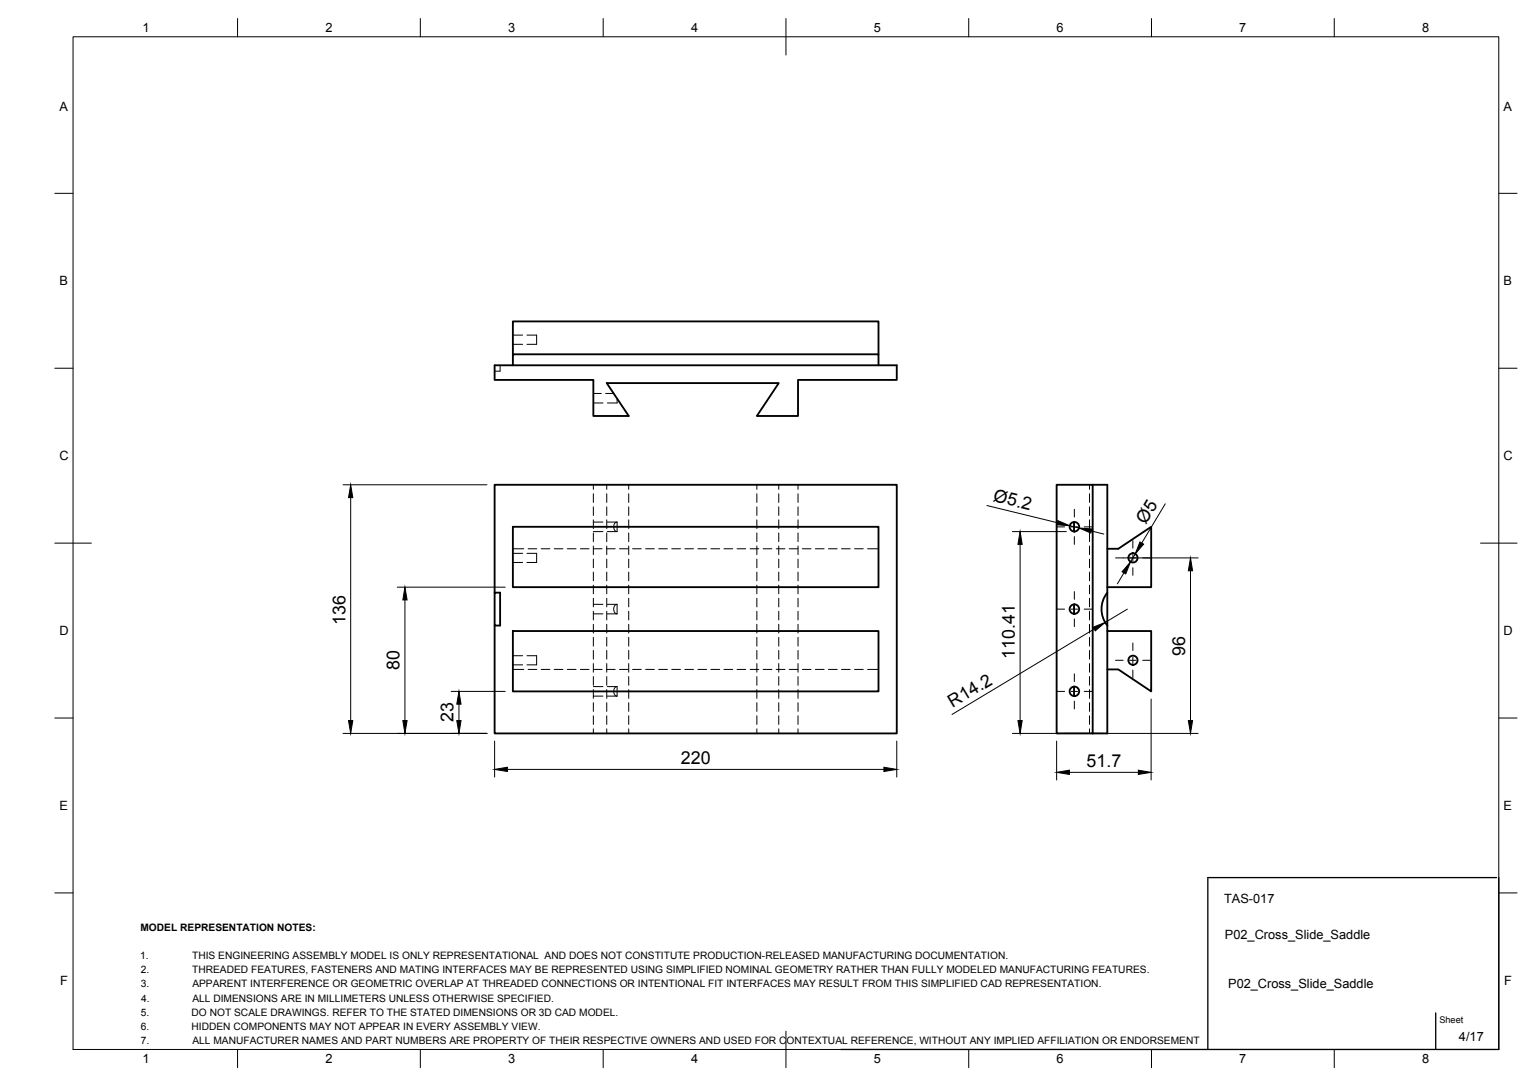
ISO-10303-21;
HEADER;
/* Generated by software containing ST-Developer
 * from STEP Tools, Inc. (www.steptools.com) 
 */

FILE_DESCRIPTION(
/* description */ ('STEP AP203'),
/* implementation_level */ '2;1');

FILE_NAME(
/* name */ 'P02_Cross_Slide_Saddle.step',
/* time_stamp */ '2026-11-15T15:04:01-08:00',
/* author */ (''),
/* organization */ (''),
/* preprocessor_version */ 'ST-DEVELOPER v20.2',
/* originating_system */ 'Autodesk Translation Framework v15.17.0.0',
/* authorisation */ '');

FILE_SCHEMA (('AUTOMOTIVE_DESIGN { 1 0 10303 214 3 1 1 }'));
ENDSEC;

DATA;
#10=MECHANICAL_DESIGN_GEOMETRIC_PRESENTATION_REPRESENTATION('',(#279,#280,#281),#16598);
#195=ELLIPSE('',#10144,3.12481110540129,2.59999999999927);
#196=ELLIPSE('',#10146,3.12481110540129,2.59999999999927);
#197=ELLIPSE('',#10149,3.12481110540191,2.59999999999976);
#198=ELLIPSE('',#10151,3.12481110540191,2.59999999999976);
#199=ELLIPSE('',#10154,3.1248111054022,2.60000000000004);
#200=ELLIPSE('',#10156,3.1248111054022,2.60000000000004);
#205=SHAPE_REPRESENTATION_RELATIONSHIP('SRR','None',#16699,#229);
#229=ADVANCED_BREP_SHAPE_REPRESENTATION('',(#253),#16575);
#253=MANIFOLD_SOLID_BREP('Body1',#9788);
#279=STYLED_ITEM('',(#16828),#9306);
#280=STYLED_ITEM('',(#16828),#9312);
#281=STYLED_ITEM('',(#16829),#253);
#310=FACE_BOUND('',#1521,.T.);
#311=FACE_BOUND('',#1522,.T.);
#312=FACE_BOUND('',#1524,.T.);
#313=FACE_BOUND('',#1525,.T.);
#314=FACE_BOUND('',#1526,.T.);
#315=FACE_BOUND('',#1535,.T.);
#316=FACE_BOUND('',#1536,.T.);
#317=FACE_BOUND('',#1537,.T.);
#318=FACE_BOUND('',#1547,.T.);
#319=FACE_BOUND('',#1554,.T.);
#474=PLANE('',#10157);
#475=PLANE('',#10158);
#476=PLANE('',#10159);
#477=PLANE('',#10160);
#478=PLANE('',#10161);
#479=PLANE('',#10162);
#480=PLANE('',#10163);
#481=PLANE('',#10164);
#482=PLANE('',#10165);
#483=PLANE('',#10166);
#484=PLANE('',#10167);
#485=PLANE('',#10168);
#486=PLANE('',#10169);
#487=PLANE('',#10170);
#488=PLANE('',#10171);
#489=PLANE('',#10172);
#490=PLANE('',#10173);
#491=PLANE('',#10174);
#492=PLANE('',#10175);
#493=PLANE('',#10176);
#494=PLANE('',#10177);
#495=PLANE('',#10178);
#496=PLANE('',#10179);
#497=PLANE('',#10180);
#498=PLANE('',#10181);
#499=PLANE('',#10182);
#500=PLANE('',#10183);
#501=PLANE('',#10184);
#502=PLANE('',#10185);
#503=PLANE('',#10186);
#504=PLANE('',#10187);
#505=PLANE('',#10188);
#959=FACE_OUTER_BOUND('',#1514,.T.);
#960=FACE_OUTER_BOUND('',#1515,.T.);
#961=FACE_OUTER_BOUND('',#1516,.T.);
#962=FACE_OUTER_BOUND('',#1517,.T.);
#963=FACE_OUTER_BOUND('',#1518,.T.);
#964=FACE_OUTER_BOUND('',#1519,.T.);
#965=FACE_OUTER_BOUND('',#1520,.T.);
#966=FACE_OUTER_BOUND('',#1523,.T.);
#967=FACE_OUTER_BOUND('',#1527,.T.);
#968=FACE_OUTER_BOUND('',#1528,.T.);
#969=FACE_OUTER_BOUND('',#1529,.T.);
#970=FACE_OUTER_BOUND('',#1530,.T.);
#971=FACE_OUTER_BOUND('',#1531,.T.);
#972=FACE_OUTER_BOUND('',#1532,.T.);
#973=FACE_OUTER_BOUND('',#1533,.T.);
#974=FACE_OUTER_BOUND('',#1534,.T.);
#975=FACE_OUTER_BOUND('',#1538,.T.);
#976=FACE_OUTER_BOUND('',#1539,.T.);
#977=FACE_OUTER_BOUND('',#1540,.T.);
#978=FACE_OUTER_BOUND('',#1541,.T.);
#979=FACE_OUTER_BOUND('',#1542,.T.);
#980=FACE_OUTER_BOUND('',#1543,.T.);
#981=FACE_OUTER_BOUND('',#1544,.T.);
#982=FACE_OUTER_BOUND('',#1545,.T.);
#983=FACE_OUTER_BOUND('',#1546,.T.);
#984=FACE_OUTER_BOUND('',#1548,.T.);
#985=FACE_OUTER_BOUND('',#1549,.T.);
#986=FACE_OUTER_BOUND('',#1550,.T.);
#987=FACE_OUTER_BOUND('',#1551,.T.);
#988=FACE_OUTER_BOUND('',#1552,.T.);
#989=FACE_OUTER_BOUND('',#1553,.T.);
#990=FACE_OUTER_BOUND('',#1555,.T.);
#991=FACE_OUTER_BOUND('',#1556,.T.);
#992=FACE_OUTER_BOUND('',#1557,.T.);
#993=FACE_OUTER_BOUND('',#1558,.T.);
#994=FACE_OUTER_BOUND('',#1559,.T.);
#995=FACE_OUTER_BOUND('',#1560,.T.);
#996=FACE_OUTER_BOUND('',#1561,.T.);
#1514=EDGE_LOOP('',(#6849,#6850,#6851,#6852));
#1515=EDGE_LOOP('',(#6853,#6854,#6855,#6856));
#1516=EDGE_LOOP('',(#6857,#6858,#6859,#6860));
#1517=EDGE_LOOP('',(#6861,#6862,#6863,#6864,#6865,#6866));
#1518=EDGE_LOOP('',(#6867,#6868,#6869,#6870,#6871,#6872));
#1519=EDGE_LOOP('',(#6873,#6874,#6875,#6876,#6877,#6878));
#1520=EDGE_LOOP('',(#6879,#6880,#6881,#6882,#6883,#6884,#6885,#6886));
#1521=EDGE_LOOP('',(#6887,#6888,#6889,#6890));
#1522=EDGE_LOOP('',(#6891,#6892,#6893,#6894));
#1523=EDGE_LOOP('',(#6895,#6896,#6897,#6898));
#1524=EDGE_LOOP('',(#6899,#6900,#6901));
#1525=EDGE_LOOP('',(#6902,#6903,#6904));
#1526=EDGE_LOOP('',(#6905,#6906,#6907));
#1527=EDGE_LOOP('',(#6908,#6909,#6910,#6911));
#1528=EDGE_LOOP('',(#6912,#6913,#6914,#6915));
#1529=EDGE_LOOP('',(#6916,#6917,#6918,#6919));
#1530=EDGE_LOOP('',(#6920,#6921,#6922,#6923));
#1531=EDGE_LOOP('',(#6924,#6925,#6926,#6927));
#1532=EDGE_LOOP('',(#6928,#6929,#6930,#6931));
#1533=EDGE_LOOP('',(#6932,#6933,#6934,#6935));
#1534=EDGE_LOOP('',(#6936,#6937,#6938,#6939));
#1535=EDGE_LOOP('',(#6940));
#1536=EDGE_LOOP('',(#6941));
#1537=EDGE_LOOP('',(#6942));
#1538=EDGE_LOOP('',(#6943,#6944,#6945,#6946));
#1539=EDGE_LOOP('',(#6947,#6948,#6949,#6950,#6951,#6952));
#1540=EDGE_LOOP('',(#6953,#6954,#6955,#6956,#6957,#6958,#6959,#6960,#6961,
#6962,#6963,#6964));
#1541=EDGE_LOOP('',(#6965,#6966,#6967,#6968,#6969,#6970,#6971,#6972,#6973,
#6974,#6975,#6976));
#1542=EDGE_LOOP('',(#6977,#6978,#6979,#6980));
#1543=EDGE_LOOP('',(#6981,#6982,#6983,#6984));
#1544=EDGE_LOOP('',(#6985,#6986,#6987,#6988));
#1545=EDGE_LOOP('',(#6989,#6990,#6991,#6992));
#1546=EDGE_LOOP('',(#6993,#6994,#6995,#6996,#6997));
#1547=EDGE_LOOP('',(#6998));
#1548=EDGE_LOOP('',(#6999,#7000,#7001,#7002,#7003));
#1549=EDGE_LOOP('',(#7004,#7005,#7006,#7007));
#1550=EDGE_LOOP('',(#7008,#7009,#7010,#7011));
#1551=EDGE_LOOP('',(#7012,#7013,#7014,#7015));
#1552=EDGE_LOOP('',(#7016,#7017,#7018,#7019));
#1553=EDGE_LOOP('',(#7020,#7021,#7022,#7023,#7024));
#1554=EDGE_LOOP('',(#7025));
#1555=EDGE_LOOP('',(#7026,#7027,#7028,#7029,#7030));
#1556=EDGE_LOOP('',(#7031,#7032));
#1557=EDGE_LOOP('',(#7033,#7034));
#1558=EDGE_LOOP('',(#7035,#7036));
#1559=EDGE_LOOP('',(#7037));
#1560=EDGE_LOOP('',(#7038));
#1561=EDGE_LOOP('',(#7039,#7040));
#2256=LINE('',#13946,#3304);
#2257=LINE('',#13949,#3305);
#2258=LINE('',#13954,#3306);
#2259=LINE('',#13960,#3307);
#2260=LINE('',#13966,#3308);
#2261=LINE('',#13976,#3309);
#2262=LINE('',#13986,#3310);
#2263=LINE('',#13993,#3311);
#2264=LINE('',#13995,#3312);
#2265=LINE('',#13997,#3313);
#2266=LINE('',#13999,#3314);
#2267=LINE('',#14001,#3315);
#2268=LINE('',#14002,#3316);
#2269=LINE('',#14005,#3317);
#2270=LINE('',#14007,#3318);
#2271=LINE('',#14009,#3319);
#2272=LINE('',#14010,#3320);
#2273=LINE('',#14013,#3321);
#2274=LINE('',#14015,#3322);
#2275=LINE('',#14017,#3323);
#2276=LINE('',#14018,#3324);
#2277=LINE('',#14022,#3325);
#2278=LINE('',#14024,#3326);
#2279=LINE('',#14026,#3327);
#2280=LINE('',#14027,#3328);
#2281=LINE('',#14028,#3329);
#2282=LINE('',#14029,#3330);
#2283=LINE('',#14030,#3331);
#2284=LINE('',#14033,#3332);
#2285=LINE('',#14035,#3333);
#2286=LINE('',#14036,#3334);
#2287=LINE('',#14039,#3335);
#2288=LINE('',#14041,#3336);
#2289=LINE('',#14042,#3337);
#2290=LINE('',#14045,#3338);
#2291=LINE('',#14047,#3339);
#2292=LINE('',#14048,#3340);
#2293=LINE('',#14051,#3341);
#2294=LINE('',#14053,#3342);
#2295=LINE('',#14054,#3343);
#2296=LINE('',#14057,#3344);
#2297=LINE('',#14059,#3345);
#2298=LINE('',#14060,#3346);
#2299=LINE('',#14062,#3347);
#2300=LINE('',#14063,#3348);
#2301=LINE('',#14066,#3349);
#2302=LINE('',#14068,#3350);
#2303=LINE('',#14069,#3351);
#2304=LINE('',#14072,#3352);
#2305=LINE('',#14074,#3353);
#2306=LINE('',#14075,#3354);
#2307=LINE('',#14078,#3355);
#2308=LINE('',#14080,#3356);
#2309=LINE('',#14081,#3357);
#2310=LINE('',#14083,#3358);
#2311=LINE('',#14084,#3359);
#2312=LINE('',#14089,#3360);
#2313=LINE('',#14091,#3361);
#2314=LINE('',#14092,#3362);
#2315=LINE('',#14095,#3363);
#2316=LINE('',#14097,#3364);
#2317=LINE('',#14098,#3365);
#2318=LINE('',#14101,#3366);
#2319=LINE('',#14103,#3367);
#2320=LINE('',#14104,#3368);
#2321=LINE('',#14106,#3369);
#2322=LINE('',#14107,#3370);
#2323=LINE('',#14112,#3371);
#2324=LINE('',#14114,#3372);
#2325=LINE('',#14115,#3373);
#2326=LINE('',#14118,#3374);
#2327=LINE('',#14120,#3375);
#2328=LINE('',#14121,#3376);
#2329=LINE('',#14124,#3377);
#2330=LINE('',#14126,#3378);
#2331=LINE('',#14127,#3379);
#2332=LINE('',#14129,#3380);
#2333=LINE('',#14130,#3381);
#3304=VECTOR('',#11166,1000.);
#3305=VECTOR('',#11169,1000.);
#3306=VECTOR('',#11174,2.5);
#3307=VECTOR('',#11181,2.5);
#3308=VECTOR('',#11188,2.6);
#3309=VECTOR('',#11199,2.6);
#3310=VECTOR('',#11210,2.6);
#3311=VECTOR('',#11219,1000.);
#3312=VECTOR('',#11220,1000.);
#3313=VECTOR('',#11221,1000.);
#3314=VECTOR('',#11222,1000.);
#3315=VECTOR('',#11223,1000.);
#3316=VECTOR('',#11224,1000.);
#3317=VECTOR('',#11225,1000.);
#3318=VECTOR('',#11226,1000.);
#3319=VECTOR('',#11227,1000.);
#3320=VECTOR('',#11228,1000.);
#3321=VECTOR('',#11229,1000.);
#3322=VECTOR('',#11230,1000.);
#3323=VECTOR('',#11231,1000.);
#3324=VECTOR('',#11232,1000.);
#3325=VECTOR('',#11235,1000.);
#3326=VECTOR('',#11236,1000.);
#3327=VECTOR('',#11237,1000.);
#3328=VECTOR('',#11238,1000.);
#3329=VECTOR('',#11239,1000.);
#3330=VECTOR('',#11240,1000.);
#3331=VECTOR('',#11241,1000.);
#3332=VECTOR('',#11244,1000.);
#3333=VECTOR('',#11245,1000.);
#3334=VECTOR('',#11246,1000.);
#3335=VECTOR('',#11249,1000.);
#3336=VECTOR('',#11250,1000.);
#3337=VECTOR('',#11251,1000.);
#3338=VECTOR('',#11254,1000.);
#3339=VECTOR('',#11255,1000.);
#3340=VECTOR('',#11256,1000.);
#3341=VECTOR('',#11259,1000.);
#3342=VECTOR('',#11260,1000.);
#3343=VECTOR('',#11261,1000.);
#3344=VECTOR('',#11264,1000.);
#3345=VECTOR('',#11265,1000.);
#3346=VECTOR('',#11266,1000.);
#3347=VECTOR('',#11269,1000.);
#3348=VECTOR('',#11270,1000.);
#3349=VECTOR('',#11273,1000.);
#3350=VECTOR('',#11274,1000.);
#3351=VECTOR('',#11275,1000.);
#3352=VECTOR('',#11278,1000.);
#3353=VECTOR('',#11279,1000.);
#3354=VECTOR('',#11280,1000.);
#3355=VECTOR('',#11283,1000.);
#3356=VECTOR('',#11284,1000.);
#3357=VECTOR('',#11285,1000.);
#3358=VECTOR('',#11288,1000.);
#3359=VECTOR('',#11289,1000.);
#3360=VECTOR('',#11296,1000.);
#3361=VECTOR('',#11297,1000.);
#3362=VECTOR('',#11298,1000.);
#3363=VECTOR('',#11301,1000.);
#3364=VECTOR('',#11302,1000.);
#3365=VECTOR('',#11303,1000.);
#3366=VECTOR('',#11306,1000.);
#3367=VECTOR('',#11307,1000.);
#3368=VECTOR('',#11308,1000.);
#3369=VECTOR('',#11311,1000.);
#3370=VECTOR('',#11312,1000.);
#3371=VECTOR('',#11319,1000.);
#3372=VECTOR('',#11320,1000.);
#3373=VECTOR('',#11321,1000.);
#3374=VECTOR('',#11324,1000.);
#3375=VECTOR('',#11325,1000.);
#3376=VECTOR('',#11326,1000.);
#3377=VECTOR('',#11329,1000.);
#3378=VECTOR('',#11330,1000.);
#3379=VECTOR('',#11331,1000.);
#3380=VECTOR('',#11334,1000.);
#3381=VECTOR('',#11335,1000.);
#4238=CIRCLE('',#10134,14.2);
#4239=CIRCLE('',#10135,14.2);
#4240=CIRCLE('',#10137,2.5);
#4241=CIRCLE('',#10138,2.5);
#4242=CIRCLE('',#10140,2.5);
#4243=CIRCLE('',#10141,2.5);
#4244=CIRCLE('',#10143,2.6);
#4245=CIRCLE('',#10145,2.6);
#4246=CIRCLE('',#10148,2.6);
#4247=CIRCLE('',#10150,2.6);
#4248=CIRCLE('',#10153,2.6);
#4249=CIRCLE('',#10155,2.6);
#4539=VERTEX_POINT('',#13942);
#4540=VERTEX_POINT('',#13943);
#4541=VERTEX_POINT('',#13945);
#4542=VERTEX_POINT('',#13947);
#4543=VERTEX_POINT('',#13951);
#4544=VERTEX_POINT('',#13953);
#4545=VERTEX_POINT('',#13957);
#4546=VERTEX_POINT('',#13959);
#4547=VERTEX_POINT('',#13963);
#4548=VERTEX_POINT('',#13965);
#4549=VERTEX_POINT('',#13967);
#4550=VERTEX_POINT('',#13969);
#4551=VERTEX_POINT('',#13973);
#4552=VERTEX_POINT('',#13975);
#4553=VERTEX_POINT('',#13977);
#4554=VERTEX_POINT('',#13979);
#4555=VERTEX_POINT('',#13983);
#4556=VERTEX_POINT('',#13985);
#4557=VERTEX_POINT('',#13987);
#4558=VERTEX_POINT('',#13989);
#4559=VERTEX_POINT('',#13994);
#4560=VERTEX_POINT('',#13996);
#4561=VERTEX_POINT('',#13998);
#4562=VERTEX_POINT('',#14000);
#4563=VERTEX_POINT('',#14003);
#4564=VERTEX_POINT('',#14004);
#4565=VERTEX_POINT('',#14006);
#4566=VERTEX_POINT('',#14008);
#4567=VERTEX_POINT('',#14011);
#4568=VERTEX_POINT('',#14012);
#4569=VERTEX_POINT('',#14014);
#4570=VERTEX_POINT('',#14016);
#4571=VERTEX_POINT('',#14020);
#4572=VERTEX_POINT('',#14021);
#4573=VERTEX_POINT('',#14023);
#4574=VERTEX_POINT('',#14025);
#4575=VERTEX_POINT('',#14032);
#4576=VERTEX_POINT('',#14034);
#4577=VERTEX_POINT('',#14038);
#4578=VERTEX_POINT('',#14040);
#4579=VERTEX_POINT('',#14044);
#4580=VERTEX_POINT('',#14046);
#4581=VERTEX_POINT('',#14050);
#4582=VERTEX_POINT('',#14052);
#4583=VERTEX_POINT('',#14056);
#4584=VERTEX_POINT('',#14058);
#4585=VERTEX_POINT('',#14065);
#4586=VERTEX_POINT('',#14067);
#4587=VERTEX_POINT('',#14071);
#4588=VERTEX_POINT('',#14073);
#4589=VERTEX_POINT('',#14077);
#4590=VERTEX_POINT('',#14079);
#4591=VERTEX_POINT('',#14088);
#4592=VERTEX_POINT('',#14090);
#4593=VERTEX_POINT('',#14094);
#4594=VERTEX_POINT('',#14096);
#4595=VERTEX_POINT('',#14100);
#4596=VERTEX_POINT('',#14102);
#4597=VERTEX_POINT('',#14111);
#4598=VERTEX_POINT('',#14113);
#4599=VERTEX_POINT('',#14117);
#4600=VERTEX_POINT('',#14119);
#4601=VERTEX_POINT('',#14123);
#4602=VERTEX_POINT('',#14125);
#5437=EDGE_CURVE('',#4539,#4540,#4238,.T.);
#5438=EDGE_CURVE('',#4540,#4541,#2256,.T.);
#5439=EDGE_CURVE('',#4542,#4541,#4239,.T.);
#5440=EDGE_CURVE('',#4542,#4539,#2257,.T.);
#5441=EDGE_CURVE('',#4543,#4543,#4240,.T.);
#5442=EDGE_CURVE('',#4543,#4544,#2258,.T.);
#5443=EDGE_CURVE('',#4544,#4544,#4241,.T.);
#5444=EDGE_CURVE('',#4545,#4545,#4242,.T.);
#5445=EDGE_CURVE('',#4545,#4546,#2259,.T.);
#5446=EDGE_CURVE('',#4546,#4546,#4243,.T.);
#5447=EDGE_CURVE('',#4547,#4547,#4244,.T.);
#5448=EDGE_CURVE('',#4547,#4548,#2260,.T.);
#5449=EDGE_CURVE('',#4548,#4549,#195,.T.);
#5450=EDGE_CURVE('',#4550,#4549,#4245,.T.);
#5451=EDGE_CURVE('',#4550,#4548,#196,.T.);
#5452=EDGE_CURVE('',#4551,#4551,#4246,.T.);
#5453=EDGE_CURVE('',#4551,#4552,#2261,.T.);
#5454=EDGE_CURVE('',#4552,#4553,#197,.T.);
#5455=EDGE_CURVE('',#4554,#4553,#4247,.T.);
#5456=EDGE_CURVE('',#4554,#4552,#198,.T.);
#5457=EDGE_CURVE('',#4555,#4555,#4248,.T.);
#5458=EDGE_CURVE('',#4555,#4556,#2262,.T.);
#5459=EDGE_CURVE('',#4556,#4557,#199,.T.);
#5460=EDGE_CURVE('',#4558,#4557,#4249,.T.);
#5461=EDGE_CURVE('',#4558,#4556,#200,.T.);
#5462=EDGE_CURVE('',#4541,#4542,#2263,.T.);
#5463=EDGE_CURVE('',#4540,#4559,#2264,.T.);
#5464=EDGE_CURVE('',#4559,#4560,#2265,.T.);
#5465=EDGE_CURVE('',#4561,#4560,#2266,.T.);
#5466=EDGE_CURVE('',#4562,#4561,#2267,.T.);
#5467=EDGE_CURVE('',#4562,#4539,#2268,.T.);
#5468=EDGE_CURVE('',#4563,#4564,#2269,.T.);
#5469=EDGE_CURVE('',#4563,#4565,#2270,.T.);
#5470=EDGE_CURVE('',#4565,#4566,#2271,.T.);
#5471=EDGE_CURVE('',#4564,#4566,#2272,.T.);
#5472=EDGE_CURVE('',#4567,#4568,#2273,.T.);
#5473=EDGE_CURVE('',#4569,#4567,#2274,.T.);
#5474=EDGE_CURVE('',#4569,#4570,#2275,.T.);
#5475=EDGE_CURVE('',#4570,#4568,#2276,.T.);
#5476=EDGE_CURVE('',#4571,#4572,#2277,.T.);
#5477=EDGE_CURVE('',#4573,#4572,#2278,.T.);
#5478=EDGE_CURVE('',#4574,#4573,#2279,.T.);
#5479=EDGE_CURVE('',#4574,#4571,#2280,.T.);
#5480=EDGE_CURVE('',#4557,#4558,#2281,.T.);
#5481=EDGE_CURVE('',#4549,#4550,#2282,.T.);
#5482=EDGE_CURVE('',#4553,#4554,#2283,.T.);
#5483=EDGE_CURVE('',#4560,#4575,#2284,.T.);
#5484=EDGE_CURVE('',#4576,#4575,#2285,.T.);
#5485=EDGE_CURVE('',#4561,#4576,#2286,.T.);
#5486=EDGE_CURVE('',#4575,#4577,#2287,.T.);
#5487=EDGE_CURVE('',#4578,#4577,#2288,.T.);
#5488=EDGE_CURVE('',#4576,#4578,#2289,.T.);
#5489=EDGE_CURVE('',#4577,#4579,#2290,.T.);
#5490=EDGE_CURVE('',#4580,#4579,#2291,.T.);
#5491=EDGE_CURVE('',#4578,#4580,#2292,.T.);
#5492=EDGE_CURVE('',#4579,#4581,#2293,.T.);
#5493=EDGE_CURVE('',#4582,#4581,#2294,.T.);
#5494=EDGE_CURVE('',#4580,#4582,#2295,.T.);
#5495=EDGE_CURVE('',#4581,#4583,#2296,.T.);
#5496=EDGE_CURVE('',#4584,#4583,#2297,.T.);
#5497=EDGE_CURVE('',#4582,#4584,#2298,.T.);
#5498=EDGE_CURVE('',#4583,#4571,#2299,.T.);
#5499=EDGE_CURVE('',#4584,#4574,#2300,.T.);
#5500=EDGE_CURVE('',#4572,#4585,#2301,.T.);
#5501=EDGE_CURVE('',#4586,#4585,#2302,.T.);
#5502=EDGE_CURVE('',#4573,#4586,#2303,.T.);
#5503=EDGE_CURVE('',#4585,#4587,#2304,.T.);
#5504=EDGE_CURVE('',#4588,#4587,#2305,.T.);
#5505=EDGE_CURVE('',#4586,#4588,#2306,.T.);
#5506=EDGE_CURVE('',#4587,#4589,#2307,.T.);
#5507=EDGE_CURVE('',#4590,#4589,#2308,.T.);
#5508=EDGE_CURVE('',#4588,#4590,#2309,.T.);
#5509=EDGE_CURVE('',#4590,#4562,#2310,.T.);
#5510=EDGE_CURVE('',#4589,#4559,#2311,.T.);
#5511=EDGE_CURVE('',#4566,#4591,#2312,.T.);
#5512=EDGE_CURVE('',#4592,#4591,#2313,.T.);
#5513=EDGE_CURVE('',#4564,#4592,#2314,.T.);
#5514=EDGE_CURVE('',#4591,#4593,#2315,.T.);
#5515=EDGE_CURVE('',#4594,#4593,#2316,.T.);
#5516=EDGE_CURVE('',#4592,#4594,#2317,.T.);
#5517=EDGE_CURVE('',#4593,#4595,#2318,.T.);
#5518=EDGE_CURVE('',#4596,#4595,#2319,.T.);
#5519=EDGE_CURVE('',#4594,#4596,#2320,.T.);
#5520=EDGE_CURVE('',#4595,#4565,#2321,.T.);
#5521=EDGE_CURVE('',#4596,#4563,#2322,.T.);
#5522=EDGE_CURVE('',#4597,#4570,#2323,.T.);
#5523=EDGE_CURVE('',#4598,#4569,#2324,.T.);
#5524=EDGE_CURVE('',#4598,#4597,#2325,.T.);
#5525=EDGE_CURVE('',#4568,#4599,#2326,.T.);
#5526=EDGE_CURVE('',#4600,#4599,#2327,.T.);
#5527=EDGE_CURVE('',#4567,#4600,#2328,.T.);
#5528=EDGE_CURVE('',#4599,#4601,#2329,.T.);
#5529=EDGE_CURVE('',#4602,#4601,#2330,.T.);
#5530=EDGE_CURVE('',#4600,#4602,#2331,.T.);
#5531=EDGE_CURVE('',#4601,#4597,#2332,.T.);
#5532=EDGE_CURVE('',#4602,#4598,#2333,.T.);
#6849=ORIENTED_EDGE('',*,*,#5437,.T.);
#6850=ORIENTED_EDGE('',*,*,#5438,.T.);
#6851=ORIENTED_EDGE('',*,*,#5439,.F.);
#6852=ORIENTED_EDGE('',*,*,#5440,.T.);
#6853=ORIENTED_EDGE('',*,*,#5441,.T.);
#6854=ORIENTED_EDGE('',*,*,#5442,.T.);
#6855=ORIENTED_EDGE('',*,*,#5443,.F.);
#6856=ORIENTED_EDGE('',*,*,#5442,.F.);
#6857=ORIENTED_EDGE('',*,*,#5444,.F.);
#6858=ORIENTED_EDGE('',*,*,#5445,.T.);
#6859=ORIENTED_EDGE('',*,*,#5446,.F.);
#6860=ORIENTED_EDGE('',*,*,#5445,.F.);
#6861=ORIENTED_EDGE('',*,*,#5447,.T.);
#6862=ORIENTED_EDGE('',*,*,#5448,.T.);
#6863=ORIENTED_EDGE('',*,*,#5449,.T.);
#6864=ORIENTED_EDGE('',*,*,#5450,.F.);
#6865=ORIENTED_EDGE('',*,*,#5451,.T.);
#6866=ORIENTED_EDGE('',*,*,#5448,.F.);
#6867=ORIENTED_EDGE('',*,*,#5452,.T.);
#6868=ORIENTED_EDGE('',*,*,#5453,.T.);
#6869=ORIENTED_EDGE('',*,*,#5454,.T.);
#6870=ORIENTED_EDGE('',*,*,#5455,.F.);
#6871=ORIENTED_EDGE('',*,*,#5456,.T.);
#6872=ORIENTED_EDGE('',*,*,#5453,.F.);
#6873=ORIENTED_EDGE('',*,*,#5457,.T.);
#6874=ORIENTED_EDGE('',*,*,#5458,.T.);
#6875=ORIENTED_EDGE('',*,*,#5459,.T.);
#6876=ORIENTED_EDGE('',*,*,#5460,.F.);
#6877=ORIENTED_EDGE('',*,*,#5461,.T.);
#6878=ORIENTED_EDGE('',*,*,#5458,.F.);
#6879=ORIENTED_EDGE('',*,*,#5440,.F.);
#6880=ORIENTED_EDGE('',*,*,#5462,.F.);
#6881=ORIENTED_EDGE('',*,*,#5438,.F.);
#6882=ORIENTED_EDGE('',*,*,#5463,.T.);
#6883=ORIENTED_EDGE('',*,*,#5464,.T.);
#6884=ORIENTED_EDGE('',*,*,#5465,.F.);
#6885=ORIENTED_EDGE('',*,*,#5466,.F.);
#6886=ORIENTED_EDGE('',*,*,#5467,.T.);
#6887=ORIENTED_EDGE('',*,*,#5468,.F.);
#6888=ORIENTED_EDGE('',*,*,#5469,.T.);
#6889=ORIENTED_EDGE('',*,*,#5470,.T.);
#6890=ORIENTED_EDGE('',*,*,#5471,.F.);
#6891=ORIENTED_EDGE('',*,*,#5472,.F.);
#6892=ORIENTED_EDGE('',*,*,#5473,.F.);
#6893=ORIENTED_EDGE('',*,*,#5474,.T.);
#6894=ORIENTED_EDGE('',*,*,#5475,.T.);
#6895=ORIENTED_EDGE('',*,*,#5476,.T.);
#6896=ORIENTED_EDGE('',*,*,#5477,.F.);
#6897=ORIENTED_EDGE('',*,*,#5478,.F.);
#6898=ORIENTED_EDGE('',*,*,#5479,.T.);
#6899=ORIENTED_EDGE('',*,*,#5461,.F.);
#6900=ORIENTED_EDGE('',*,*,#5480,.F.);
#6901=ORIENTED_EDGE('',*,*,#5459,.F.);
#6902=ORIENTED_EDGE('',*,*,#5451,.F.);
#6903=ORIENTED_EDGE('',*,*,#5481,.F.);
#6904=ORIENTED_EDGE('',*,*,#5449,.F.);
#6905=ORIENTED_EDGE('',*,*,#5456,.F.);
#6906=ORIENTED_EDGE('',*,*,#5482,.F.);
#6907=ORIENTED_EDGE('',*,*,#5454,.F.);
#6908=ORIENTED_EDGE('',*,*,#5483,.T.);
#6909=ORIENTED_EDGE('',*,*,#5484,.F.);
#6910=ORIENTED_EDGE('',*,*,#5485,.F.);
#6911=ORIENTED_EDGE('',*,*,#5465,.T.);
#6912=ORIENTED_EDGE('',*,*,#5486,.T.);
#6913=ORIENTED_EDGE('',*,*,#5487,.F.);
#6914=ORIENTED_EDGE('',*,*,#5488,.F.);
#6915=ORIENTED_EDGE('',*,*,#5484,.T.);
#6916=ORIENTED_EDGE('',*,*,#5489,.T.);
#6917=ORIENTED_EDGE('',*,*,#5490,.F.);
#6918=ORIENTED_EDGE('',*,*,#5491,.F.);
#6919=ORIENTED_EDGE('',*,*,#5487,.T.);
#6920=ORIENTED_EDGE('',*,*,#5492,.T.);
#6921=ORIENTED_EDGE('',*,*,#5493,.F.);
#6922=ORIENTED_EDGE('',*,*,#5494,.F.);
#6923=ORIENTED_EDGE('',*,*,#5490,.T.);
#6924=ORIENTED_EDGE('',*,*,#5495,.T.);
#6925=ORIENTED_EDGE('',*,*,#5496,.F.);
#6926=ORIENTED_EDGE('',*,*,#5497,.F.);
#6927=ORIENTED_EDGE('',*,*,#5493,.T.);
#6928=ORIENTED_EDGE('',*,*,#5498,.T.);
#6929=ORIENTED_EDGE('',*,*,#5479,.F.);
#6930=ORIENTED_EDGE('',*,*,#5499,.F.);
#6931=ORIENTED_EDGE('',*,*,#5496,.T.);
#6932=ORIENTED_EDGE('',*,*,#5500,.T.);
#6933=ORIENTED_EDGE('',*,*,#5501,.F.);
#6934=ORIENTED_EDGE('',*,*,#5502,.F.);
#6935=ORIENTED_EDGE('',*,*,#5477,.T.);
#6936=ORIENTED_EDGE('',*,*,#5503,.T.);
#6937=ORIENTED_EDGE('',*,*,#5504,.F.);
#6938=ORIENTED_EDGE('',*,*,#5505,.F.);
#6939=ORIENTED_EDGE('',*,*,#5501,.T.);
#6940=ORIENTED_EDGE('',*,*,#5447,.F.);
#6941=ORIENTED_EDGE('',*,*,#5452,.F.);
#6942=ORIENTED_EDGE('',*,*,#5457,.F.);
#6943=ORIENTED_EDGE('',*,*,#5506,.T.);
#6944=ORIENTED_EDGE('',*,*,#5507,.F.);
#6945=ORIENTED_EDGE('',*,*,#5508,.F.);
#6946=ORIENTED_EDGE('',*,*,#5504,.T.);
#6947=ORIENTED_EDGE('',*,*,#5437,.F.);
#6948=ORIENTED_EDGE('',*,*,#5467,.F.);
#6949=ORIENTED_EDGE('',*,*,#5509,.F.);
#6950=ORIENTED_EDGE('',*,*,#5507,.T.);
#6951=ORIENTED_EDGE('',*,*,#5510,.T.);
#6952=ORIENTED_EDGE('',*,*,#5463,.F.);
#6953=ORIENTED_EDGE('',*,*,#5485,.T.);
#6954=ORIENTED_EDGE('',*,*,#5488,.T.);
#6955=ORIENTED_EDGE('',*,*,#5491,.T.);
#6956=ORIENTED_EDGE('',*,*,#5494,.T.);
#6957=ORIENTED_EDGE('',*,*,#5497,.T.);
#6958=ORIENTED_EDGE('',*,*,#5499,.T.);
#6959=ORIENTED_EDGE('',*,*,#5478,.T.);
#6960=ORIENTED_EDGE('',*,*,#5502,.T.);
#6961=ORIENTED_EDGE('',*,*,#5505,.T.);
#6962=ORIENTED_EDGE('',*,*,#5508,.T.);
#6963=ORIENTED_EDGE('',*,*,#5509,.T.);
#6964=ORIENTED_EDGE('',*,*,#5466,.T.);
#6965=ORIENTED_EDGE('',*,*,#5483,.F.);
#6966=ORIENTED_EDGE('',*,*,#5464,.F.);
#6967=ORIENTED_EDGE('',*,*,#5510,.F.);
#6968=ORIENTED_EDGE('',*,*,#5506,.F.);
#6969=ORIENTED_EDGE('',*,*,#5503,.F.);
#6970=ORIENTED_EDGE('',*,*,#5500,.F.);
#6971=ORIENTED_EDGE('',*,*,#5476,.F.);
#6972=ORIENTED_EDGE('',*,*,#5498,.F.);
#6973=ORIENTED_EDGE('',*,*,#5495,.F.);
#6974=ORIENTED_EDGE('',*,*,#5492,.F.);
#6975=ORIENTED_EDGE('',*,*,#5489,.F.);
#6976=ORIENTED_EDGE('',*,*,#5486,.F.);
#6977=ORIENTED_EDGE('',*,*,#5511,.T.);
#6978=ORIENTED_EDGE('',*,*,#5512,.F.);
#6979=ORIENTED_EDGE('',*,*,#5513,.F.);
#6980=ORIENTED_EDGE('',*,*,#5471,.T.);
#6981=ORIENTED_EDGE('',*,*,#5514,.T.);
#6982=ORIENTED_EDGE('',*,*,#5515,.F.);
#6983=ORIENTED_EDGE('',*,*,#5516,.F.);
#6984=ORIENTED_EDGE('',*,*,#5512,.T.);
#6985=ORIENTED_EDGE('',*,*,#5517,.T.);
#6986=ORIENTED_EDGE('',*,*,#5518,.F.);
#6987=ORIENTED_EDGE('',*,*,#5519,.F.);
#6988=ORIENTED_EDGE('',*,*,#5515,.T.);
#6989=ORIENTED_EDGE('',*,*,#5520,.T.);
#6990=ORIENTED_EDGE('',*,*,#5469,.F.);
#6991=ORIENTED_EDGE('',*,*,#5521,.F.);
#6992=ORIENTED_EDGE('',*,*,#5518,.T.);
#6993=ORIENTED_EDGE('',*,*,#5513,.T.);
#6994=ORIENTED_EDGE('',*,*,#5516,.T.);
#6995=ORIENTED_EDGE('',*,*,#5519,.T.);
#6996=ORIENTED_EDGE('',*,*,#5521,.T.);
#6997=ORIENTED_EDGE('',*,*,#5468,.T.);
#6998=ORIENTED_EDGE('',*,*,#5441,.F.);
#6999=ORIENTED_EDGE('',*,*,#5511,.F.);
#7000=ORIENTED_EDGE('',*,*,#5470,.F.);
#7001=ORIENTED_EDGE('',*,*,#5520,.F.);
#7002=ORIENTED_EDGE('',*,*,#5517,.F.);
#7003=ORIENTED_EDGE('',*,*,#5514,.F.);
#7004=ORIENTED_EDGE('',*,*,#5522,.T.);
#7005=ORIENTED_EDGE('',*,*,#5474,.F.);
#7006=ORIENTED_EDGE('',*,*,#5523,.F.);
#7007=ORIENTED_EDGE('',*,*,#5524,.T.);
#7008=ORIENTED_EDGE('',*,*,#5525,.T.);
#7009=ORIENTED_EDGE('',*,*,#5526,.F.);
#7010=ORIENTED_EDGE('',*,*,#5527,.F.);
#7011=ORIENTED_EDGE('',*,*,#5472,.T.);
#7012=ORIENTED_EDGE('',*,*,#5528,.T.);
#7013=ORIENTED_EDGE('',*,*,#5529,.F.);
#7014=ORIENTED_EDGE('',*,*,#5530,.F.);
#7015=ORIENTED_EDGE('',*,*,#5526,.T.);
#7016=ORIENTED_EDGE('',*,*,#5531,.T.);
#7017=ORIENTED_EDGE('',*,*,#5524,.F.);
#7018=ORIENTED_EDGE('',*,*,#5532,.F.);
#7019=ORIENTED_EDGE('',*,*,#5529,.T.);
#7020=ORIENTED_EDGE('',*,*,#5523,.T.);
#7021=ORIENTED_EDGE('',*,*,#5473,.T.);
#7022=ORIENTED_EDGE('',*,*,#5527,.T.);
#7023=ORIENTED_EDGE('',*,*,#5530,.T.);
#7024=ORIENTED_EDGE('',*,*,#5532,.T.);
#7025=ORIENTED_EDGE('',*,*,#5444,.T.);
#7026=ORIENTED_EDGE('',*,*,#5522,.F.);
#7027=ORIENTED_EDGE('',*,*,#5531,.F.);
#7028=ORIENTED_EDGE('',*,*,#5528,.F.);
#7029=ORIENTED_EDGE('',*,*,#5525,.F.);
#7030=ORIENTED_EDGE('',*,*,#5475,.F.);
#7031=ORIENTED_EDGE('',*,*,#5480,.T.);
#7032=ORIENTED_EDGE('',*,*,#5460,.T.);
#7033=ORIENTED_EDGE('',*,*,#5482,.T.);
#7034=ORIENTED_EDGE('',*,*,#5455,.T.);
#7035=ORIENTED_EDGE('',*,*,#5481,.T.);
#7036=ORIENTED_EDGE('',*,*,#5450,.T.);
#7037=ORIENTED_EDGE('',*,*,#5446,.T.);
#7038=ORIENTED_EDGE('',*,*,#5443,.T.);
#7039=ORIENTED_EDGE('',*,*,#5462,.T.);
#7040=ORIENTED_EDGE('',*,*,#5439,.T.);
#9172=CYLINDRICAL_SURFACE('',#10133,14.2);
#9173=CYLINDRICAL_SURFACE('',#10136,2.5);
#9174=CYLINDRICAL_SURFACE('',#10139,2.5);
#9175=CYLINDRICAL_SURFACE('',#10142,2.6);
#9176=CYLINDRICAL_SURFACE('',#10147,2.6);
#9177=CYLINDRICAL_SURFACE('',#10152,2.6);
#9284=ADVANCED_FACE('',(#959),#9172,.F.);
#9285=ADVANCED_FACE('',(#960),#9173,.F.);
#9286=ADVANCED_FACE('',(#961),#9174,.F.);
#9287=ADVANCED_FACE('',(#962),#9175,.F.);
#9288=ADVANCED_FACE('',(#963),#9176,.F.);
#9289=ADVANCED_FACE('',(#964),#9177,.F.);
#9290=ADVANCED_FACE('',(#965,#310,#311),#474,.F.);
#9291=ADVANCED_FACE('',(#966,#312,#313,#314),#475,.F.);
#9292=ADVANCED_FACE('',(#967),#476,.F.);
#9293=ADVANCED_FACE('',(#968),#477,.F.);
#9294=ADVANCED_FACE('',(#969),#478,.F.);
#9295=ADVANCED_FACE('',(#970),#479,.F.);
#9296=ADVANCED_FACE('',(#971),#480,.F.);
#9297=ADVANCED_FACE('',(#972),#481,.F.);
#9298=ADVANCED_FACE('',(#973),#482,.F.);
#9299=ADVANCED_FACE('',(#974,#315,#316,#317),#483,.F.);
#9300=ADVANCED_FACE('',(#975),#484,.F.);
#9301=ADVANCED_FACE('',(#976),#485,.F.);
#9302=ADVANCED_FACE('',(#977),#486,.T.);
#9303=ADVANCED_FACE('',(#978),#487,.F.);
#9304=ADVANCED_FACE('',(#979),#488,.F.);
#9305=ADVANCED_FACE('',(#980),#489,.F.);
#9306=ADVANCED_FACE('',(#981),#490,.F.);
#9307=ADVANCED_FACE('',(#982),#491,.F.);
#9308=ADVANCED_FACE('',(#983,#318),#492,.F.);
#9309=ADVANCED_FACE('',(#984),#493,.T.);
#9310=ADVANCED_FACE('',(#985),#494,.F.);
#9311=ADVANCED_FACE('',(#986),#495,.F.);
#9312=ADVANCED_FACE('',(#987),#496,.F.);
#9313=ADVANCED_FACE('',(#988),#497,.F.);
#9314=ADVANCED_FACE('',(#989,#319),#498,.T.);
#9315=ADVANCED_FACE('',(#990),#499,.F.);
#9316=ADVANCED_FACE('',(#991),#500,.T.);
#9317=ADVANCED_FACE('',(#992),#501,.T.);
#9318=ADVANCED_FACE('',(#993),#502,.T.);
#9319=ADVANCED_FACE('',(#994),#503,.T.);
#9320=ADVANCED_FACE('',(#995),#504,.T.);
#9321=ADVANCED_FACE('',(#996),#505,.T.);
#9788=CLOSED_SHELL('',(#9284,#9285,#9286,#9287,#9288,#9289,#9290,#9291,
#9292,#9293,#9294,#9295,#9296,#9297,#9298,#9299,#9300,#9301,#9302,#9303,
#9304,#9305,#9306,#9307,#9308,#9309,#9310,#9311,#9312,#9313,#9314,#9315,
#9316,#9317,#9318,#9319,#9320,#9321));
#10132=AXIS2_PLACEMENT_3D('',#13940,#11160,#11161);
#10133=AXIS2_PLACEMENT_3D('',#13941,#11162,#11163);
#10134=AXIS2_PLACEMENT_3D('',#13944,#11164,#11165);
#10135=AXIS2_PLACEMENT_3D('',#13948,#11167,#11168);
#10136=AXIS2_PLACEMENT_3D('',#13950,#11170,#11171);
#10137=AXIS2_PLACEMENT_3D('',#13952,#11172,#11173);
#10138=AXIS2_PLACEMENT_3D('',#13955,#11175,#11176);
#10139=AXIS2_PLACEMENT_3D('',#13956,#11177,#11178);
#10140=AXIS2_PLACEMENT_3D('',#13958,#11179,#11180);
#10141=AXIS2_PLACEMENT_3D('',#13961,#11182,#11183);
#10142=AXIS2_PLACEMENT_3D('',#13962,#11184,#11185);
#10143=AXIS2_PLACEMENT_3D('',#13964,#11186,#11187);
#10144=AXIS2_PLACEMENT_3D('',#13968,#11189,#11190);
#10145=AXIS2_PLACEMENT_3D('',#13970,#11191,#11192);
#10146=AXIS2_PLACEMENT_3D('',#13971,#11193,#11194);
#10147=AXIS2_PLACEMENT_3D('',#13972,#11195,#11196);
#10148=AXIS2_PLACEMENT_3D('',#13974,#11197,#11198);
#10149=AXIS2_PLACEMENT_3D('',#13978,#11200,#11201);
#10150=AXIS2_PLACEMENT_3D('',#13980,#11202,#11203);
#10151=AXIS2_PLACEMENT_3D('',#13981,#11204,#11205);
#10152=AXIS2_PLACEMENT_3D('',#13982,#11206,#11207);
#10153=AXIS2_PLACEMENT_3D('',#13984,#11208,#11209);
#10154=AXIS2_PLACEMENT_3D('',#13988,#11211,#11212);
#10155=AXIS2_PLACEMENT_3D('',#13990,#11213,#11214);
#10156=AXIS2_PLACEMENT_3D('',#13991,#11215,#11216);
#10157=AXIS2_PLACEMENT_3D('',#13992,#11217,#11218);
#10158=AXIS2_PLACEMENT_3D('',#14019,#11233,#11234);
#10159=AXIS2_PLACEMENT_3D('',#14031,#11242,#11243);
#10160=AXIS2_PLACEMENT_3D('',#14037,#11247,#11248);
#10161=AXIS2_PLACEMENT_3D('',#14043,#11252,#11253);
#10162=AXIS2_PLACEMENT_3D('',#14049,#11257,#11258);
#10163=AXIS2_PLACEMENT_3D('',#14055,#11262,#11263);
#10164=AXIS2_PLACEMENT_3D('',#14061,#11267,#11268);
#10165=AXIS2_PLACEMENT_3D('',#14064,#11271,#11272);
#10166=AXIS2_PLACEMENT_3D('',#14070,#11276,#11277);
#10167=AXIS2_PLACEMENT_3D('',#14076,#11281,#11282);
#10168=AXIS2_PLACEMENT_3D('',#14082,#11286,#11287);
#10169=AXIS2_PLACEMENT_3D('',#14085,#11290,#11291);
#10170=AXIS2_PLACEMENT_3D('',#14086,#11292,#11293);
#10171=AXIS2_PLACEMENT_3D('',#14087,#11294,#11295);
#10172=AXIS2_PLACEMENT_3D('',#14093,#11299,#11300);
#10173=AXIS2_PLACEMENT_3D('',#14099,#11304,#11305);
#10174=AXIS2_PLACEMENT_3D('',#14105,#11309,#11310);
#10175=AXIS2_PLACEMENT_3D('',#14108,#11313,#11314);
#10176=AXIS2_PLACEMENT_3D('',#14109,#11315,#11316);
#10177=AXIS2_PLACEMENT_3D('',#14110,#11317,#11318);
#10178=AXIS2_PLACEMENT_3D('',#14116,#11322,#11323);
#10179=AXIS2_PLACEMENT_3D('',#14122,#11327,#11328);
#10180=AXIS2_PLACEMENT_3D('',#14128,#11332,#11333);
#10181=AXIS2_PLACEMENT_3D('',#14131,#11336,#11337);
#10182=AXIS2_PLACEMENT_3D('',#14132,#11338,#11339);
#10183=AXIS2_PLACEMENT_3D('',#14133,#11340,#11341);
#10184=AXIS2_PLACEMENT_3D('',#14134,#11342,#11343);
#10185=AXIS2_PLACEMENT_3D('',#14135,#11344,#11345);
#10186=AXIS2_PLACEMENT_3D('',#14136,#11346,#11347);
#10187=AXIS2_PLACEMENT_3D('',#14137,#11348,#11349);
#10188=AXIS2_PLACEMENT_3D('',#14138,#11350,#11351);
#11160=DIRECTION('axis',(0.,0.,1.));
#11161=DIRECTION('refdir',(1.,0.,0.));
#11162=DIRECTION('center_axis',(0.,-1.,0.));
#11163=DIRECTION('ref_axis',(0.,0.,-1.));
#11164=DIRECTION('center_axis',(0.,1.,0.));
#11165=DIRECTION('ref_axis',(2.66453525910038E-15,0.,-1.));
#11166=DIRECTION('',(0.,-1.,0.));
#11167=DIRECTION('center_axis',(0.,1.,0.));
#11168=DIRECTION('ref_axis',(0.,0.,1.));
#11169=DIRECTION('',(0.,1.,0.));
#11170=DIRECTION('center_axis',(0.,-1.,0.));
#11171=DIRECTION('ref_axis',(0.,0.,-1.));
#11172=DIRECTION('center_axis',(0.,1.,0.));
#11173=DIRECTION('ref_axis',(0.,0.,-1.));
#11174=DIRECTION('',(0.,-1.,0.));
#11175=DIRECTION('center_axis',(0.,1.,0.));
#11176=DIRECTION('ref_axis',(0.,0.,1.));
#11177=DIRECTION('center_axis',(0.,-1.,0.));
#11178=DIRECTION('ref_axis',(0.,0.,-1.));
#11179=DIRECTION('center_axis',(0.,-1.,0.));
#11180=DIRECTION('ref_axis',(0.,0.,1.));
#11181=DIRECTION('',(0.,-1.,0.));
#11182=DIRECTION('center_axis',(0.,1.,0.));
#11183=DIRECTION('ref_axis',(0.,0.,1.));
#11184=DIRECTION('center_axis',(0.,-1.,0.));
#11185=DIRECTION('ref_axis',(0.,0.,-1.));
#11186=DIRECTION('center_axis',(0.,1.,0.));
#11187=DIRECTION('ref_axis',(0.,0.,-1.));
#11188=DIRECTION('',(0.,-1.,0.));
#11189=DIRECTION('center_axis',(3.03770030380451E-15,-0.832050294337844,
0.554700196225228));
#11190=DIRECTION('ref_axis',(-6.45395818566141E-13,-0.554700196225228,-0.832050294337844));
#11191=DIRECTION('center_axis',(0.,1.,0.));
#11192=DIRECTION('ref_axis',(0.,0.,1.));
#11193=DIRECTION('center_axis',(3.03770030380451E-15,-0.832050294337844,
0.554700196225228));
#11194=DIRECTION('ref_axis',(-6.45395818566141E-13,-0.554700196225228,-0.832050294337844));
#11195=DIRECTION('center_axis',(0.,-1.,0.));
#11196=DIRECTION('ref_axis',(0.,0.,-1.));
#11197=DIRECTION('center_axis',(0.,1.,0.));
#11198=DIRECTION('ref_axis',(0.,0.,-1.));
#11199=DIRECTION('',(0.,-1.,0.));
#11200=DIRECTION('center_axis',(-2.10302328724925E-15,-0.832050294337843,
0.554700196225231));
#11201=DIRECTION('ref_axis',(-1.7015761927577E-13,-0.55470019622523,-0.832050294337843));
#11202=DIRECTION('center_axis',(0.,1.,0.));
#11203=DIRECTION('ref_axis',(0.,0.,1.));
#11204=DIRECTION('center_axis',(-2.10302328724925E-15,-0.832050294337843,
0.554700196225231));
#11205=DIRECTION('ref_axis',(-1.7015761927577E-13,-0.55470019622523,-0.832050294337843));
#11206=DIRECTION('center_axis',(0.,-1.,0.));
#11207=DIRECTION('ref_axis',(0.,0.,-1.));
#11208=DIRECTION('center_axis',(0.,1.,0.));
#11209=DIRECTION('ref_axis',(0.,0.,-1.));
#11210=DIRECTION('',(0.,-1.,0.));
#11211=DIRECTION('center_axis',(3.0377003038045E-15,-0.832050294337844,
0.554700196225229));
#11212=DIRECTION('ref_axis',(4.33987867344828E-14,-0.554700196225228,-0.832050294337844));
#11213=DIRECTION('center_axis',(0.,1.,0.));
#11214=DIRECTION('ref_axis',(0.,0.,1.));
#11215=DIRECTION('center_axis',(3.0377003038045E-15,-0.832050294337844,
0.554700196225229));
#11216=DIRECTION('ref_axis',(4.33987867344828E-14,-0.554700196225228,-0.832050294337844));
#11217=DIRECTION('center_axis',(0.,0.,-1.));
#11218=DIRECTION('ref_axis',(-1.,0.,0.));
#11219=DIRECTION('',(1.,0.,0.));
#11220=DIRECTION('',(-1.,0.,0.));
#11221=DIRECTION('',(0.,-1.,0.));
#11222=DIRECTION('',(-1.,0.,0.));
#11223=DIRECTION('',(0.,-1.,0.));
#11224=DIRECTION('',(-1.,0.,0.));
#11225=DIRECTION('',(-1.,0.,0.));
#11226=DIRECTION('',(0.,-1.,0.));
#11227=DIRECTION('',(-1.,0.,0.));
#11228=DIRECTION('',(0.,-1.,0.));
#11229=DIRECTION('',(0.,-1.,0.));
#11230=DIRECTION('',(-1.,0.,0.));
#11231=DIRECTION('',(0.,-1.,0.));
#11232=DIRECTION('',(-1.,0.,0.));
#11233=DIRECTION('center_axis',(0.,0.832050294337844,-0.554700196225229));
#11234=DIRECTION('ref_axis',(0.,0.554700196225229,0.832050294337844));
#11235=DIRECTION('',(0.,-0.554700196225229,-0.832050294337844));
#11236=DIRECTION('',(-1.,0.,0.));
#11237=DIRECTION('',(0.,-0.554700196225229,-0.832050294337844));
#11238=DIRECTION('',(-1.,0.,0.));
#11239=DIRECTION('',(1.,0.,0.));
#11240=DIRECTION('',(1.,0.,0.));
#11241=DIRECTION('',(1.,0.,0.));
#11242=DIRECTION('center_axis',(0.,1.,0.));
#11243=DIRECTION('ref_axis',(0.,0.,1.));
#11244=DIRECTION('',(0.,0.,-1.));
#11245=DIRECTION('',(-1.,0.,0.));
#11246=DIRECTION('',(0.,0.,-1.));
#11247=DIRECTION('center_axis',(0.,0.,1.));
#11248=DIRECTION('ref_axis',(1.,0.,0.));
#11249=DIRECTION('',(0.,1.,0.));
#11250=DIRECTION('',(-1.,0.,0.));
#11251=DIRECTION('',(0.,1.,0.));
#11252=DIRECTION('center_axis',(0.,1.,0.));
#11253=DIRECTION('ref_axis',(0.,0.,1.));
#11254=DIRECTION('',(0.,0.,-1.));
#11255=DIRECTION('',(-1.,0.,0.));
#11256=DIRECTION('',(0.,0.,-1.));
#11257=DIRECTION('center_axis',(0.,0.,1.));
#11258=DIRECTION('ref_axis',(1.,0.,0.));
#11259=DIRECTION('',(0.,1.,0.));
#11260=DIRECTION('',(-1.,0.,0.));
#11261=DIRECTION('',(0.,1.,0.));
#11262=DIRECTION('center_axis',(0.,-0.832050294337844,-0.554700196225229));
#11263=DIRECTION('ref_axis',(0.,0.554700196225229,-0.832050294337843));
#11264=DIRECTION('',(0.,-0.554700196225229,0.832050294337843));
#11265=DIRECTION('',(-1.,0.,0.));
#11266=DIRECTION('',(0.,-0.554700196225229,0.832050294337843));
#11267=DIRECTION('center_axis',(0.,0.,1.));
#11268=DIRECTION('ref_axis',(1.,0.,0.));
#11269=DIRECTION('',(0.,1.,0.));
#11270=DIRECTION('',(0.,1.,0.));
#11271=DIRECTION('center_axis',(0.,0.,1.));
#11272=DIRECTION('ref_axis',(1.,0.,0.));
#11273=DIRECTION('',(0.,1.,0.));
#11274=DIRECTION('',(-1.,0.,0.));
#11275=DIRECTION('',(0.,1.,0.));
#11276=DIRECTION('center_axis',(0.,-1.,0.));
#11277=DIRECTION('ref_axis',(0.,0.,-1.));
#11278=DIRECTION('',(0.,0.,1.));
#11279=DIRECTION('',(-1.,0.,0.));
#11280=DIRECTION('',(0.,0.,1.));
#11281=DIRECTION('center_axis',(0.,0.,1.));
#11282=DIRECTION('ref_axis',(1.,0.,0.));
#11283=DIRECTION('',(0.,1.,0.));
#11284=DIRECTION('',(-1.,0.,0.));
#11285=DIRECTION('',(0.,1.,0.));
#11286=DIRECTION('center_axis',(0.,-1.,0.));
#11287=DIRECTION('ref_axis',(0.,0.,-1.));
#11288=DIRECTION('',(0.,0.,1.));
#11289=DIRECTION('',(0.,0.,1.));
#11290=DIRECTION('center_axis',(1.,0.,0.));
#11291=DIRECTION('ref_axis',(0.,0.,-1.));
#11292=DIRECTION('center_axis',(1.,0.,0.));
#11293=DIRECTION('ref_axis',(0.,0.,-1.));
#11294=DIRECTION('center_axis',(1.,0.,0.));
#11295=DIRECTION('ref_axis',(0.,0.,-1.));
#11296=DIRECTION('',(0.,0.,1.));
#11297=DIRECTION('',(0.,-1.,0.));
#11298=DIRECTION('',(0.,0.,1.));
#11299=DIRECTION('center_axis',(0.832050294337844,0.,0.554700196225229));
#11300=DIRECTION('ref_axis',(0.554700196225229,0.,-0.832050294337844));
#11301=DIRECTION('',(-0.554700196225229,0.,0.832050294337844));
#11302=DIRECTION('',(0.,-1.,0.));
#11303=DIRECTION('',(-0.554700196225229,0.,0.832050294337844));
#11304=DIRECTION('center_axis',(0.,0.,-1.));
#11305=DIRECTION('ref_axis',(-1.,0.,0.));
#11306=DIRECTION('',(1.,0.,0.));
#11307=DIRECTION('',(0.,-1.,0.));
#11308=DIRECTION('',(1.,0.,0.));
#11309=DIRECTION('center_axis',(-1.,0.,0.));
#11310=DIRECTION('ref_axis',(0.,0.,1.));
#11311=DIRECTION('',(0.,0.,-1.));
#11312=DIRECTION('',(0.,0.,-1.));
#11313=DIRECTION('center_axis',(0.,-1.,0.));
#11314=DIRECTION('ref_axis',(0.,0.,-1.));
#11315=DIRECTION('center_axis',(0.,-1.,0.));
#11316=DIRECTION('ref_axis',(0.,0.,-1.));
#11317=DIRECTION('center_axis',(-1.,0.,0.));
#11318=DIRECTION('ref_axis',(0.,0.,1.));
#11319=DIRECTION('',(0.,0.,-1.));
#11320=DIRECTION('',(0.,0.,-1.));
#11321=DIRECTION('',(0.,-1.,0.));
#11322=DIRECTION('center_axis',(1.,0.,0.));
#11323=DIRECTION('ref_axis',(0.,0.,-1.));
#11324=DIRECTION('',(0.,0.,1.));
#11325=DIRECTION('',(0.,-1.,0.));
#11326=DIRECTION('',(0.,0.,1.));
#11327=DIRECTION('center_axis',(0.,0.,-1.));
#11328=DIRECTION('ref_axis',(-1.,0.,0.));
#11329=DIRECTION('',(1.,0.,0.));
#11330=DIRECTION('',(0.,-1.,0.));
#11331=DIRECTION('',(1.,0.,0.));
#11332=DIRECTION('center_axis',(-0.832050294337844,0.,0.554700196225229));
#11333=DIRECTION('ref_axis',(0.554700196225229,0.,0.832050294337844));
#11334=DIRECTION('',(-0.554700196225229,0.,-0.832050294337844));
#11335=DIRECTION('',(-0.554700196225229,0.,-0.832050294337844));
#11336=DIRECTION('center_axis',(0.,1.,0.));
#11337=DIRECTION('ref_axis',(0.,0.,1.));
#11338=DIRECTION('center_axis',(0.,1.,0.));
#11339=DIRECTION('ref_axis',(0.,0.,1.));
#11340=DIRECTION('center_axis',(0.,1.,0.));
#11341=DIRECTION('ref_axis',(0.,0.,1.));
#11342=DIRECTION('center_axis',(0.,1.,0.));
#11343=DIRECTION('ref_axis',(0.,0.,1.));
#11344=DIRECTION('center_axis',(0.,1.,0.));
#11345=DIRECTION('ref_axis',(0.,0.,1.));
#11346=DIRECTION('center_axis',(0.,1.,0.));
#11347=DIRECTION('ref_axis',(0.,0.,1.));
#11348=DIRECTION('center_axis',(0.,1.,0.));
#11349=DIRECTION('ref_axis',(0.,0.,1.));
#11350=DIRECTION('center_axis',(0.,1.,0.));
#11351=DIRECTION('ref_axis',(0.,0.,1.));
#13940=CARTESIAN_POINT('',(0.,0.,0.));
#13941=CARTESIAN_POINT('Origin',(0.,111.,55.));
#13942=CARTESIAN_POINT('',(8.97997772825745,110.,44.));
#13943=CARTESIAN_POINT('',(-8.97997772825745,110.,44.));
#13944=CARTESIAN_POINT('Origin',(0.,110.,55.));
#13945=CARTESIAN_POINT('',(-8.97997772825745,107.,44.));
#13946=CARTESIAN_POINT('',(-8.97997772825745,111.,44.));
#13947=CARTESIAN_POINT('',(8.97997772825745,107.,44.));
#13948=CARTESIAN_POINT('Origin',(0.,107.,55.));
#13949=CARTESIAN_POINT('',(8.97997772825745,111.,44.));
#13950=CARTESIAN_POINT('Origin',(-28.,101.,58.));
#13951=CARTESIAN_POINT('',(-28.,100.,60.5));
#13952=CARTESIAN_POINT('Origin',(-28.,100.,58.));
#13953=CARTESIAN_POINT('',(-28.,87.,60.5));
#13954=CARTESIAN_POINT('',(-28.,101.,60.5));
#13955=CARTESIAN_POINT('Origin',(-28.,87.,58.));
#13956=CARTESIAN_POINT('Origin',(28.,101.,58.));
#13957=CARTESIAN_POINT('',(28.,100.,60.5));
#13958=CARTESIAN_POINT('Origin',(28.,100.,58.));
#13959=CARTESIAN_POINT('',(28.,87.,60.5));
#13960=CARTESIAN_POINT('',(28.,101.,60.5));
#13961=CARTESIAN_POINT('Origin',(28.,87.,58.));
#13962=CARTESIAN_POINT('Origin',(-45.,58.,26.));
#13963=CARTESIAN_POINT('',(-45.,56.,28.6));
#13964=CARTESIAN_POINT('Origin',(-45.,56.,26.));
#13965=CARTESIAN_POINT('',(-45.,44.85,28.6));
#13966=CARTESIAN_POINT('',(-45.,58.,28.6));
#13967=CARTESIAN_POINT('',(-47.5941038915202,43.,25.825));
#13968=CARTESIAN_POINT('Origin',(-45.0000000000008,43.1166666666671,26.0000000000007));
#13969=CARTESIAN_POINT('',(-42.4058961084799,43.,25.825));
#13970=CARTESIAN_POINT('Origin',(-45.,43.,26.));
#13971=CARTESIAN_POINT('Origin',(-45.0000000000008,43.1166666666671,26.0000000000007));
#13972=CARTESIAN_POINT('Origin',(0.,58.,26.));
#13973=CARTESIAN_POINT('',(-3.18408167778312E-16,56.,28.6));
#13974=CARTESIAN_POINT('Origin',(0.,56.,26.));
#13975=CARTESIAN_POINT('',(-3.18408167778385E-16,44.85,28.6));
#13976=CARTESIAN_POINT('',(-3.18408167778312E-16,58.,28.6));
#13977=CARTESIAN_POINT('',(-2.59410389152015,43.,25.825));
#13978=CARTESIAN_POINT('Origin',(-2.41519961368208E-13,43.1166666666668,
26.0000000000002));
#13979=CARTESIAN_POINT('',(2.59410389152015,43.,25.825));
#13980=CARTESIAN_POINT('Origin',(0.,43.,26.));
#13981=CARTESIAN_POINT('Origin',(-2.41519961368208E-13,43.1166666666668,
26.0000000000002));
#13982=CARTESIAN_POINT('Origin',(45.,58.,26.));
#13983=CARTESIAN_POINT('',(45.,56.,28.6));
#13984=CARTESIAN_POINT('Origin',(45.,56.,26.));
#13985=CARTESIAN_POINT('',(45.,44.85,28.6));
#13986=CARTESIAN_POINT('',(45.,58.,28.6));
#13987=CARTESIAN_POINT('',(42.4058961084799,43.,25.825));
#13988=CARTESIAN_POINT('Origin',(45.,43.1166666666666,25.9999999999999));
#13989=CARTESIAN_POINT('',(47.5941038915202,43.,25.825));
#13990=CARTESIAN_POINT('Origin',(45.,43.,26.));
#13991=CARTESIAN_POINT('Origin',(45.,43.1166666666666,25.9999999999999));
#13992=CARTESIAN_POINT('Origin',(68.,110.,44.));
#13993=CARTESIAN_POINT('',(68.,107.,44.));
#13994=CARTESIAN_POINT('',(-68.,110.,44.));
#13995=CARTESIAN_POINT('',(68.,110.,44.));
#13996=CARTESIAN_POINT('',(-68.,-110.,44.));
#13997=CARTESIAN_POINT('',(-68.,110.,44.));
#13998=CARTESIAN_POINT('',(68.,-110.,44.));
#13999=CARTESIAN_POINT('',(68.,-110.,44.));
#14000=CARTESIAN_POINT('',(68.,110.,44.));
#14001=CARTESIAN_POINT('',(68.,110.,44.));
#14002=CARTESIAN_POINT('',(68.,110.,44.));
#14003=CARTESIAN_POINT('',(-12.,100.,44.));
#14004=CARTESIAN_POINT('',(-33.,100.,44.));
#14005=CARTESIAN_POINT('',(-33.,100.,44.));
#14006=CARTESIAN_POINT('',(-12.,-100.,44.));
#14007=CARTESIAN_POINT('',(-12.,100.,44.));
#14008=CARTESIAN_POINT('',(-33.,-100.,44.));
#14009=CARTESIAN_POINT('',(-33.,-100.,44.));
#14010=CARTESIAN_POINT('',(-33.,100.,44.));
#14011=CARTESIAN_POINT('',(12.,100.,44.));
#14012=CARTESIAN_POINT('',(12.,-100.,44.));
#14013=CARTESIAN_POINT('',(12.,100.,44.));
#14014=CARTESIAN_POINT('',(33.,100.,44.));
#14015=CARTESIAN_POINT('',(33.,100.,44.));
#14016=CARTESIAN_POINT('',(33.,-100.,44.));
#14017=CARTESIAN_POINT('',(33.,100.,44.));
#14018=CARTESIAN_POINT('',(33.,-100.,44.));
#14019=CARTESIAN_POINT('Origin',(68.,48.65,34.3));
#14020=CARTESIAN_POINT('',(-68.,48.65,34.3));
#14021=CARTESIAN_POINT('',(-68.,36.65,16.3));
#14022=CARTESIAN_POINT('',(-68.,48.65,34.3));
#14023=CARTESIAN_POINT('',(68.,36.65,16.3));
#14024=CARTESIAN_POINT('',(68.,36.65,16.3));
#14025=CARTESIAN_POINT('',(68.,48.65,34.3));
#14026=CARTESIAN_POINT('',(68.,48.65,34.3));
#14027=CARTESIAN_POINT('',(68.,48.65,34.3));
#14028=CARTESIAN_POINT('',(68.,43.,25.825));
#14029=CARTESIAN_POINT('',(68.,43.,25.825));
#14030=CARTESIAN_POINT('',(68.,43.,25.825));
#14031=CARTESIAN_POINT('Origin',(68.,-110.,44.));
#14032=CARTESIAN_POINT('',(-68.,-110.,36.));
#14033=CARTESIAN_POINT('',(-68.,-110.,44.));
#14034=CARTESIAN_POINT('',(68.,-110.,36.));
#14035=CARTESIAN_POINT('',(68.,-110.,36.));
#14036=CARTESIAN_POINT('',(68.,-110.,44.));
#14037=CARTESIAN_POINT('Origin',(68.,-110.,36.));
#14038=CARTESIAN_POINT('',(-68.,-56.,36.));
#14039=CARTESIAN_POINT('',(-68.,-110.,36.));
#14040=CARTESIAN_POINT('',(68.,-56.,36.));
#14041=CARTESIAN_POINT('',(68.,-56.,36.));
#14042=CARTESIAN_POINT('',(68.,-110.,36.));
#14043=CARTESIAN_POINT('Origin',(68.,-56.,36.));
#14044=CARTESIAN_POINT('',(-68.,-56.,16.3));
#14045=CARTESIAN_POINT('',(-68.,-56.,36.));
#14046=CARTESIAN_POINT('',(68.,-56.,16.3));
#14047=CARTESIAN_POINT('',(68.,-56.,16.3));
#14048=CARTESIAN_POINT('',(68.,-56.,36.));
#14049=CARTESIAN_POINT('Origin',(68.,-56.,16.3));
#14050=CARTESIAN_POINT('',(-68.,-33.45,16.3));
#14051=CARTESIAN_POINT('',(-68.,-56.,16.3));
#14052=CARTESIAN_POINT('',(68.,-33.45,16.3));
#14053=CARTESIAN_POINT('',(68.,-33.45,16.3));
#14054=CARTESIAN_POINT('',(68.,-56.,16.3));
#14055=CARTESIAN_POINT('Origin',(68.,-33.45,16.3));
#14056=CARTESIAN_POINT('',(-68.,-45.45,34.3));
#14057=CARTESIAN_POINT('',(-68.,-33.45,16.3));
#14058=CARTESIAN_POINT('',(68.,-45.45,34.3));
#14059=CARTESIAN_POINT('',(68.,-45.45,34.3));
#14060=CARTESIAN_POINT('',(68.,-33.45,16.3));
#14061=CARTESIAN_POINT('Origin',(68.,-45.45,34.3));
#14062=CARTESIAN_POINT('',(-68.,-45.45,34.3));
#14063=CARTESIAN_POINT('',(68.,-45.45,34.3));
#14064=CARTESIAN_POINT('Origin',(68.,36.65,16.3));
#14065=CARTESIAN_POINT('',(-68.,56.,16.3));
#14066=CARTESIAN_POINT('',(-68.,36.65,16.3));
#14067=CARTESIAN_POINT('',(68.,56.,16.3));
#14068=CARTESIAN_POINT('',(68.,56.,16.3));
#14069=CARTESIAN_POINT('',(68.,36.65,16.3));
#14070=CARTESIAN_POINT('Origin',(68.,56.,16.3));
#14071=CARTESIAN_POINT('',(-68.,56.,36.));
#14072=CARTESIAN_POINT('',(-68.,56.,16.3));
#14073=CARTESIAN_POINT('',(68.,56.,36.));
#14074=CARTESIAN_POINT('',(68.,56.,36.));
#14075=CARTESIAN_POINT('',(68.,56.,16.3));
#14076=CARTESIAN_POINT('Origin',(68.,56.,36.));
#14077=CARTESIAN_POINT('',(-68.,110.,36.));
#14078=CARTESIAN_POINT('',(-68.,56.,36.));
#14079=CARTESIAN_POINT('',(68.,110.,36.));
#14080=CARTESIAN_POINT('',(68.,110.,36.));
#14081=CARTESIAN_POINT('',(68.,56.,36.));
#14082=CARTESIAN_POINT('Origin',(68.,110.,36.));
#14083=CARTESIAN_POINT('',(68.,110.,36.));
#14084=CARTESIAN_POINT('',(-68.,110.,36.));
#14085=CARTESIAN_POINT('Origin',(68.,0.,0.));
#14086=CARTESIAN_POINT('Origin',(-68.,0.,0.));
#14087=CARTESIAN_POINT('Origin',(-33.,100.,50.));
#14088=CARTESIAN_POINT('',(-33.,-100.,50.));
#14089=CARTESIAN_POINT('',(-33.,-100.,50.));
#14090=CARTESIAN_POINT('',(-33.,100.,50.));
#14091=CARTESIAN_POINT('',(-33.,100.,50.));
#14092=CARTESIAN_POINT('',(-33.,100.,50.));
#14093=CARTESIAN_POINT('Origin',(-45.,100.,68.));
#14094=CARTESIAN_POINT('',(-45.,-100.,68.));
#14095=CARTESIAN_POINT('',(-45.,-100.,68.));
#14096=CARTESIAN_POINT('',(-45.,100.,68.));
#14097=CARTESIAN_POINT('',(-45.,100.,68.));
#14098=CARTESIAN_POINT('',(-45.,100.,68.));
#14099=CARTESIAN_POINT('Origin',(-12.,100.,68.));
#14100=CARTESIAN_POINT('',(-12.,-100.,68.));
#14101=CARTESIAN_POINT('',(-12.,-100.,68.));
#14102=CARTESIAN_POINT('',(-12.,100.,68.));
#14103=CARTESIAN_POINT('',(-12.,100.,68.));
#14104=CARTESIAN_POINT('',(-12.,100.,68.));
#14105=CARTESIAN_POINT('Origin',(-12.,100.,44.));
#14106=CARTESIAN_POINT('',(-12.,-100.,44.));
#14107=CARTESIAN_POINT('',(-12.,100.,44.));
#14108=CARTESIAN_POINT('Origin',(0.,100.,0.));
#14109=CARTESIAN_POINT('Origin',(0.,-100.,0.));
#14110=CARTESIAN_POINT('Origin',(33.,100.,50.));
#14111=CARTESIAN_POINT('',(33.,-100.,50.));
#14112=CARTESIAN_POINT('',(33.,-100.,50.));
#14113=CARTESIAN_POINT('',(33.,100.,50.));
#14114=CARTESIAN_POINT('',(33.,100.,50.));
#14115=CARTESIAN_POINT('',(33.,100.,50.));
#14116=CARTESIAN_POINT('Origin',(12.,100.,44.));
#14117=CARTESIAN_POINT('',(12.,-100.,68.));
#14118=CARTESIAN_POINT('',(12.,-100.,44.));
#14119=CARTESIAN_POINT('',(12.,100.,68.));
#14120=CARTESIAN_POINT('',(12.,100.,68.));
#14121=CARTESIAN_POINT('',(12.,100.,44.));
#14122=CARTESIAN_POINT('Origin',(12.,100.,68.));
#14123=CARTESIAN_POINT('',(45.,-100.,68.));
#14124=CARTESIAN_POINT('',(12.,-100.,68.));
#14125=CARTESIAN_POINT('',(45.,100.,68.));
#14126=CARTESIAN_POINT('',(45.,100.,68.));
#14127=CARTESIAN_POINT('',(12.,100.,68.));
#14128=CARTESIAN_POINT('Origin',(45.,100.,68.));
#14129=CARTESIAN_POINT('',(45.,-100.,68.));
#14130=CARTESIAN_POINT('',(45.,100.,68.));
#14131=CARTESIAN_POINT('Origin',(0.,100.,0.));
#14132=CARTESIAN_POINT('Origin',(0.,-100.,0.));
#14133=CARTESIAN_POINT('Origin',(45.,43.,26.));
#14134=CARTESIAN_POINT('Origin',(0.,43.,26.));
#14135=CARTESIAN_POINT('Origin',(-45.,43.,26.));
#14136=CARTESIAN_POINT('Origin',(28.,87.,58.));
#14137=CARTESIAN_POINT('Origin',(-28.,87.,58.));
#14138=CARTESIAN_POINT('Origin',(0.,107.,55.));
#16549=UNCERTAINTY_MEASURE_WITH_UNIT(LENGTH_MEASURE(0.01),#16599,
'DISTANCE_ACCURACY_VALUE',
'Maximum model space distance between geometric entities at asserted c
onnectivities');
#16572=UNCERTAINTY_MEASURE_WITH_UNIT(LENGTH_MEASURE(0.01),#16599,
'DISTANCE_ACCURACY_VALUE',
'Maximum model space distance between geometric entities at asserted c
onnectivities');
#16575=(
GEOMETRIC_REPRESENTATION_CONTEXT(3)
GLOBAL_UNCERTAINTY_ASSIGNED_CONTEXT((#16549))
GLOBAL_UNIT_ASSIGNED_CONTEXT((#16599,#16601,#16602))
REPRESENTATION_CONTEXT('','3D')
);
#16598=(
GEOMETRIC_REPRESENTATION_CONTEXT(3)
GLOBAL_UNCERTAINTY_ASSIGNED_CONTEXT((#16572))
GLOBAL_UNIT_ASSIGNED_CONTEXT((#16599,#16601,#16602))
REPRESENTATION_CONTEXT('','3D')
);
#16599=(
LENGTH_UNIT()
NAMED_UNIT(*)
SI_UNIT(.MILLI.,.METRE.)
);
#16601=(
NAMED_UNIT(*)
PLANE_ANGLE_UNIT()
SI_UNIT($,.RADIAN.)
);
#16602=(
NAMED_UNIT(*)
SI_UNIT($,.STERADIAN.)
SOLID_ANGLE_UNIT()
);
#16605=SHAPE_DEFINITION_REPRESENTATION(#16630,#16699);
#16630=PRODUCT_DEFINITION_SHAPE('',$,#16725);
#16699=SHAPE_REPRESENTATION('',(#10132),#16575);
#16722=PRODUCT_DEFINITION_CONTEXT('part definition',#16799,'design');
#16725=PRODUCT_DEFINITION('P02_Cross_Slide_Saddle',
'P02_Cross_Slide_Saddle',#16750,#16722);
#16750=PRODUCT_DEFINITION_FORMATION('',$,#16803);
#16799=APPLICATION_CONTEXT(
'Core Data for Automotive Mechanical Design Process');
#16800=PRODUCT_CONTEXT('part definition',#16799,'mechanical');
#16803=PRODUCT('P02_Cross_Slide_Saddle','P02_Cross_Slide_Saddle',$,(#16800));
#16828=PRESENTATION_STYLE_ASSIGNMENT((#16837));
#16829=PRESENTATION_STYLE_ASSIGNMENT((#16838));
#16837=SURFACE_STYLE_USAGE(.BOTH.,#16846);
#16838=SURFACE_STYLE_USAGE(.BOTH.,#16847);
#16846=SURFACE_SIDE_STYLE('',(#16855));
#16847=SURFACE_SIDE_STYLE('',(#16856));
#16855=SURFACE_STYLE_FILL_AREA(#16864);
#16856=SURFACE_STYLE_FILL_AREA(#16865);
#16864=FILL_AREA_STYLE('Opaque(147,158,163)',(#16873));
#16865=FILL_AREA_STYLE('Light Gray',(#16874));
#16873=FILL_AREA_STYLE_COLOUR('Opaque(147,158,163)',#16882);
#16874=FILL_AREA_STYLE_COLOUR('Light Gray',#16883);
#16882=COLOUR_RGB('Opaque(147,158,163)',0.576470588235294,0.619607843137255,
0.63921568627451);
#16883=COLOUR_RGB('Light Gray',0.827450980392157,0.827450980392157,0.827450980392157);
ENDSEC;
END-ISO-10303-21;
